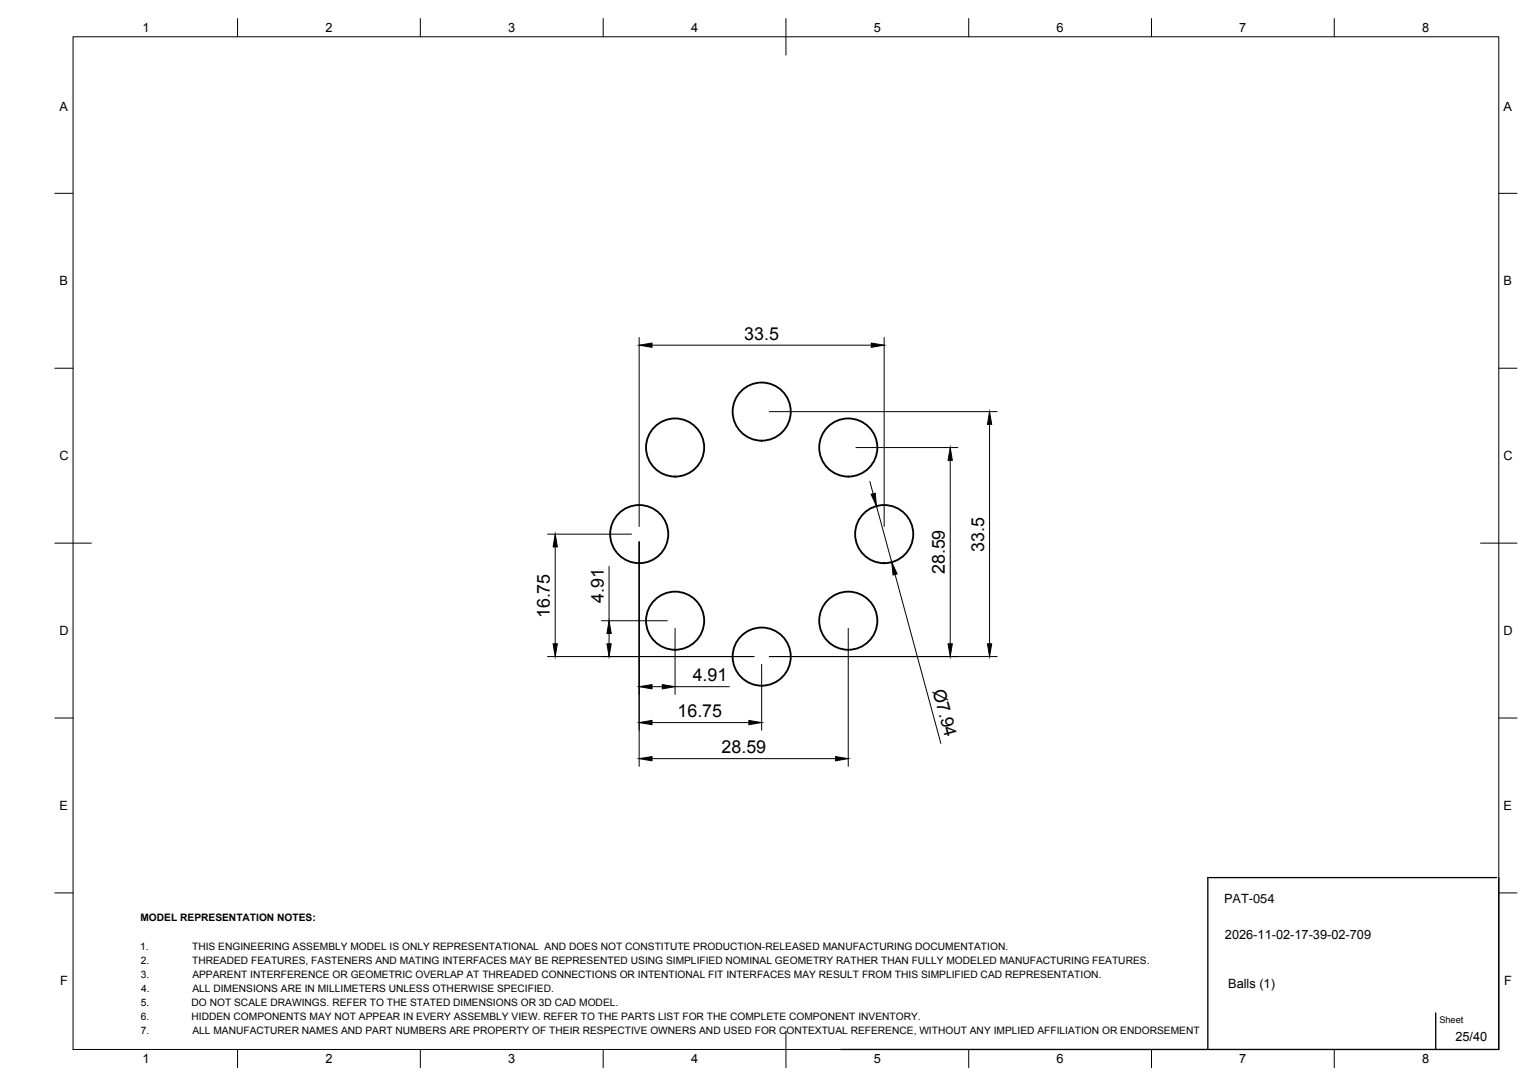
ISO-10303-21;
HEADER;
/* Generated by software containing ST-Developer
 * from STEP Tools, Inc. (www.steptools.com) 
 */

FILE_DESCRIPTION(
/* description */ ('PAT-054'),
/* implementation_level */ '2;1');

FILE_NAME(
/* name */ 'Balls (1).step',
/* time_stamp */ '2026-10-29T16:38:13-07:00',
/* author */ (''),
/* organization */ (''),
/* preprocessor_version */ 'ST-DEVELOPER v20.2',
/* originating_system */ 'Autodesk Translation Framework v15.17.0.0',
/* authorisation */ '');

FILE_SCHEMA (('AUTOMOTIVE_DESIGN { 1 0 10303 214 3 1 1 }'));
ENDSEC;

DATA;
#10=MECHANICAL_DESIGN_GEOMETRIC_PRESENTATION_REPRESENTATION('',(#922,#923,#924,#925,#926,#927,#928,#929),#33981);
#761=SPHERICAL_SURFACE('',#14041,0.3969);
#762=SPHERICAL_SURFACE('',#14043,0.3969);
#763=SPHERICAL_SURFACE('',#14045,0.3969);
#764=SPHERICAL_SURFACE('',#14047,0.3969);
#765=SPHERICAL_SURFACE('',#14049,0.3969);
#766=SPHERICAL_SURFACE('',#14051,0.3969);
#767=SPHERICAL_SURFACE('',#14053,0.3969);
#768=SPHERICAL_SURFACE('',#14055,0.3969);
#827=SHAPE_REPRESENTATION_RELATIONSHIP('SRR','None',#34202,#871);
#871=ADVANCED_BREP_SHAPE_REPRESENTATION('',(#981,#982,#983,#984,#985,#986,
#987,#988),#33950);
#922=STYLED_ITEM('',(#34517),#981);
#923=STYLED_ITEM('',(#34517),#982);
#924=STYLED_ITEM('',(#34517),#983);
#925=STYLED_ITEM('',(#34517),#984);
#926=STYLED_ITEM('',(#34517),#985);
#927=STYLED_ITEM('',(#34517),#986);
#928=STYLED_ITEM('',(#34517),#987);
#929=STYLED_ITEM('',(#34517),#988);
#981=MANIFOLD_SOLID_BREP('Body1',#13033);
#982=MANIFOLD_SOLID_BREP('Body2',#13034);
#983=MANIFOLD_SOLID_BREP('Body3',#13035);
#984=MANIFOLD_SOLID_BREP('Body4',#13036);
#985=MANIFOLD_SOLID_BREP('Body5',#13037);
#986=MANIFOLD_SOLID_BREP('Body6',#13038);
#987=MANIFOLD_SOLID_BREP('Body7',#13039);
#988=MANIFOLD_SOLID_BREP('Body8',#13040);
#1792=FACE_OUTER_BOUND('',#2644,.T.);
#1793=FACE_OUTER_BOUND('',#2645,.T.);
#1794=FACE_OUTER_BOUND('',#2646,.T.);
#1795=FACE_OUTER_BOUND('',#2647,.T.);
#1796=FACE_OUTER_BOUND('',#2648,.T.);
#1797=FACE_OUTER_BOUND('',#2649,.T.);
#1798=FACE_OUTER_BOUND('',#2650,.T.);
#1799=FACE_OUTER_BOUND('',#2651,.T.);
#2644=EDGE_LOOP('',(#9489,#9490));
#2645=EDGE_LOOP('',(#9491,#9492));
#2646=EDGE_LOOP('',(#9493,#9494));
#2647=EDGE_LOOP('',(#9495,#9496));
#2648=EDGE_LOOP('',(#9497,#9498));
#2649=EDGE_LOOP('',(#9499,#9500));
#2650=EDGE_LOOP('',(#9501,#9502));
#2651=EDGE_LOOP('',(#9503,#9504));
#5344=CIRCLE('',#14042,0.3969);
#5345=CIRCLE('',#14044,0.3969);
#5346=CIRCLE('',#14046,0.3969);
#5347=CIRCLE('',#14048,0.3969);
#5348=CIRCLE('',#14050,0.3969);
#5349=CIRCLE('',#14052,0.3969);
#5350=CIRCLE('',#14054,0.3969);
#5351=CIRCLE('',#14056,0.3969);
#5910=VERTEX_POINT('',#19864);
#5911=VERTEX_POINT('',#19865);
#5912=VERTEX_POINT('',#19868);
#5913=VERTEX_POINT('',#19869);
#5914=VERTEX_POINT('',#19872);
#5915=VERTEX_POINT('',#19873);
#5916=VERTEX_POINT('',#19876);
#5917=VERTEX_POINT('',#19877);
#5918=VERTEX_POINT('',#19880);
#5919=VERTEX_POINT('',#19881);
#5920=VERTEX_POINT('',#19884);
#5921=VERTEX_POINT('',#19885);
#5922=VERTEX_POINT('',#19888);
#5923=VERTEX_POINT('',#19889);
#5924=VERTEX_POINT('',#19892);
#5925=VERTEX_POINT('',#19893);
#7244=EDGE_CURVE('',#5910,#5911,#5344,.T.);
#7245=EDGE_CURVE('',#5912,#5913,#5345,.T.);
#7246=EDGE_CURVE('',#5914,#5915,#5346,.T.);
#7247=EDGE_CURVE('',#5916,#5917,#5347,.T.);
#7248=EDGE_CURVE('',#5918,#5919,#5348,.T.);
#7249=EDGE_CURVE('',#5920,#5921,#5349,.T.);
#7250=EDGE_CURVE('',#5922,#5923,#5350,.T.);
#7251=EDGE_CURVE('',#5924,#5925,#5351,.T.);
#9489=ORIENTED_EDGE('',*,*,#7244,.T.);
#9490=ORIENTED_EDGE('',*,*,#7244,.F.);
#9491=ORIENTED_EDGE('',*,*,#7245,.T.);
#9492=ORIENTED_EDGE('',*,*,#7245,.F.);
#9493=ORIENTED_EDGE('',*,*,#7246,.T.);
#9494=ORIENTED_EDGE('',*,*,#7246,.F.);
#9495=ORIENTED_EDGE('',*,*,#7247,.T.);
#9496=ORIENTED_EDGE('',*,*,#7247,.F.);
#9497=ORIENTED_EDGE('',*,*,#7248,.T.);
#9498=ORIENTED_EDGE('',*,*,#7248,.F.);
#9499=ORIENTED_EDGE('',*,*,#7249,.T.);
#9500=ORIENTED_EDGE('',*,*,#7249,.F.);
#9501=ORIENTED_EDGE('',*,*,#7250,.T.);
#9502=ORIENTED_EDGE('',*,*,#7250,.F.);
#9503=ORIENTED_EDGE('',*,*,#7251,.T.);
#9504=ORIENTED_EDGE('',*,*,#7251,.F.);
#12504=ADVANCED_FACE('',(#1792),#761,.T.);
#12505=ADVANCED_FACE('',(#1793),#762,.T.);
#12506=ADVANCED_FACE('',(#1794),#763,.T.);
#12507=ADVANCED_FACE('',(#1795),#764,.T.);
#12508=ADVANCED_FACE('',(#1796),#765,.T.);
#12509=ADVANCED_FACE('',(#1797),#766,.T.);
#12510=ADVANCED_FACE('',(#1798),#767,.T.);
#12511=ADVANCED_FACE('',(#1799),#768,.T.);
#13033=CLOSED_SHELL('',(#12504));
#13034=CLOSED_SHELL('',(#12505));
#13035=CLOSED_SHELL('',(#12506));
#13036=CLOSED_SHELL('',(#12507));
#13037=CLOSED_SHELL('',(#12508));
#13038=CLOSED_SHELL('',(#12509));
#13039=CLOSED_SHELL('',(#12510));
#13040=CLOSED_SHELL('',(#12511));
#14040=AXIS2_PLACEMENT_3D('',#19862,#16099,#16100);
#14041=AXIS2_PLACEMENT_3D('',#19863,#16101,#16102);
#14042=AXIS2_PLACEMENT_3D('',#19866,#16103,#16104);
#14043=AXIS2_PLACEMENT_3D('',#19867,#16105,#16106);
#14044=AXIS2_PLACEMENT_3D('',#19870,#16107,#16108);
#14045=AXIS2_PLACEMENT_3D('',#19871,#16109,#16110);
#14046=AXIS2_PLACEMENT_3D('',#19874,#16111,#16112);
#14047=AXIS2_PLACEMENT_3D('',#19875,#16113,#16114);
#14048=AXIS2_PLACEMENT_3D('',#19878,#16115,#16116);
#14049=AXIS2_PLACEMENT_3D('',#19879,#16117,#16118);
#14050=AXIS2_PLACEMENT_3D('',#19882,#16119,#16120);
#14051=AXIS2_PLACEMENT_3D('',#19883,#16121,#16122);
#14052=AXIS2_PLACEMENT_3D('',#19886,#16123,#16124);
#14053=AXIS2_PLACEMENT_3D('',#19887,#16125,#16126);
#14054=AXIS2_PLACEMENT_3D('',#19890,#16127,#16128);
#14055=AXIS2_PLACEMENT_3D('',#19891,#16129,#16130);
#14056=AXIS2_PLACEMENT_3D('',#19894,#16131,#16132);
#16099=DIRECTION('axis',(0.,0.,1.));
#16100=DIRECTION('refdir',(1.,0.,0.));
#16101=DIRECTION('center_axis',(0.,0.,1.));
#16102=DIRECTION('ref_axis',(1.,0.,0.));
#16103=DIRECTION('center_axis',(1.22464679914735E-16,-1.,0.));
#16104=DIRECTION('ref_axis',(-1.,-1.22464679914735E-16,0.));
#16105=DIRECTION('center_axis',(0.707106781186548,0.,0.707106781186548));
#16106=DIRECTION('ref_axis',(0.707106781186548,0.,-0.707106781186548));
#16107=DIRECTION('center_axis',(8.65956056235493E-17,-1.,-8.65956056235493E-17));
#16108=DIRECTION('ref_axis',(-0.707106781186548,-1.22464679914735E-16,0.707106781186548));
#16109=DIRECTION('center_axis',(1.,0.,0.));
#16110=DIRECTION('ref_axis',(6.12323399573677E-17,0.,-1.));
#16111=DIRECTION('center_axis',(7.49879891330929E-33,-1.,-1.22464679914735E-16));
#16112=DIRECTION('ref_axis',(-6.12323399573677E-17,-1.22464679914735E-16,
1.));
#16113=DIRECTION('center_axis',(0.707106781186548,0.,-0.707106781186548));
#16114=DIRECTION('ref_axis',(-0.707106781186548,0.,-0.707106781186548));
#16115=DIRECTION('center_axis',(-8.65956056235493E-17,-1.,-8.65956056235493E-17));
#16116=DIRECTION('ref_axis',(0.707106781186548,-1.22464679914735E-16,0.707106781186548));
#16117=DIRECTION('center_axis',(0.,0.,-1.));
#16118=DIRECTION('ref_axis',(-1.,0.,-1.22464679914735E-16));
#16119=DIRECTION('center_axis',(-1.22464679914735E-16,-1.,-1.49975978266186E-32));
#16120=DIRECTION('ref_axis',(1.,-1.22464679914735E-16,1.22464679914735E-16));
#16121=DIRECTION('center_axis',(-0.707106781186548,0.,-0.707106781186548));
#16122=DIRECTION('ref_axis',(-0.707106781186548,0.,0.707106781186548));
#16123=DIRECTION('center_axis',(-8.65956056235493E-17,-1.,8.65956056235493E-17));
#16124=DIRECTION('ref_axis',(0.707106781186548,-1.22464679914735E-16,-0.707106781186548));
#16125=DIRECTION('center_axis',(-1.,0.,0.));
#16126=DIRECTION('ref_axis',(-1.83697019872103E-16,0.,1.));
#16127=DIRECTION('center_axis',(-2.24963967399279E-32,-1.,1.22464679914735E-16));
#16128=DIRECTION('ref_axis',(1.83697019872103E-16,-1.22464679914735E-16,
-1.));
#16129=DIRECTION('center_axis',(-0.707106781186548,0.,0.707106781186548));
#16130=DIRECTION('ref_axis',(0.707106781186548,0.,0.707106781186548));
#16131=DIRECTION('center_axis',(8.65956056235493E-17,-1.,8.65956056235494E-17));
#16132=DIRECTION('ref_axis',(-0.707106781186548,-1.22464679914735E-16,-0.707106781186548));
#19862=CARTESIAN_POINT('',(0.,0.,0.));
#19863=CARTESIAN_POINT('Origin',(1.675,0.,0.));
#19864=CARTESIAN_POINT('',(1.675,-2.97627328869245E-33,0.3969));
#19865=CARTESIAN_POINT('',(1.675,-2.97627328869245E-33,-0.3969));
#19866=CARTESIAN_POINT('Origin',(1.675,0.,0.));
#19867=CARTESIAN_POINT('Origin',(1.18440385848747,0.,-1.18440385848747));
#19868=CARTESIAN_POINT('',(1.46505453994041,3.1867025333467E-33,-0.903753177034526));
#19869=CARTESIAN_POINT('',(0.903753177034527,-9.13924911073161E-33,-1.46505453994041));
#19870=CARTESIAN_POINT('Origin',(1.18440385848747,0.,-1.18440385848747));
#19871=CARTESIAN_POINT('Origin',(1.02564169428591E-16,0.,-1.675));
#19872=CARTESIAN_POINT('',(0.3969,-2.97627328869246E-33,-1.675));
#19873=CARTESIAN_POINT('',(-0.3969,-2.97627328869245E-33,-1.675));
#19874=CARTESIAN_POINT('Origin',(1.02564169428591E-16,0.,-1.675));
#19875=CARTESIAN_POINT('Origin',(-1.18440385848747,0.,-1.18440385848747));
#19876=CARTESIAN_POINT('',(-0.903753177034526,3.1867025333467E-33,-1.46505453994041));
#19877=CARTESIAN_POINT('',(-1.46505453994041,-9.13924911073161E-33,-0.903753177034527));
#19878=CARTESIAN_POINT('Origin',(-1.18440385848747,0.,-1.18440385848747));
#19879=CARTESIAN_POINT('Origin',(-1.675,0.,-2.05128338857182E-16));
#19880=CARTESIAN_POINT('',(-1.675,-2.97627328869246E-33,-0.3969));
#19881=CARTESIAN_POINT('',(-1.675,-2.97627328869245E-33,0.3969));
#19882=CARTESIAN_POINT('Origin',(-1.675,0.,-2.05128338857182E-16));
#19883=CARTESIAN_POINT('Origin',(-1.18440385848747,0.,1.18440385848747));
#19884=CARTESIAN_POINT('',(-1.46505453994041,6.26819044436628E-33,0.903753177034526));
#19885=CARTESIAN_POINT('',(-0.903753177034527,-1.22207370217512E-32,1.46505453994041));
#19886=CARTESIAN_POINT('Origin',(-1.18440385848747,0.,1.18440385848747));
#19887=CARTESIAN_POINT('Origin',(-3.07692508285772E-16,0.,1.675));
#19888=CARTESIAN_POINT('',(-0.3969,-2.97627328869246E-33,1.675));
#19889=CARTESIAN_POINT('',(0.396899999999999,-2.97627328869245E-33,1.675));
#19890=CARTESIAN_POINT('Origin',(-3.07692508285772E-16,0.,1.675));
#19891=CARTESIAN_POINT('Origin',(1.18440385848747,0.,1.18440385848747));
#19892=CARTESIAN_POINT('',(0.903753177034526,9.34967835538585E-33,1.46505453994041));
#19893=CARTESIAN_POINT('',(1.46505453994041,-1.53022249327708E-32,0.903753177034527));
#19894=CARTESIAN_POINT('Origin',(1.18440385848747,0.,1.18440385848747));
#33898=UNCERTAINTY_MEASURE_WITH_UNIT(LENGTH_MEASURE(0.001),#33982,
'DISTANCE_ACCURACY_VALUE',
'Maximum model space distance between geometric entities at asserted c
onnectivities');
#33929=UNCERTAINTY_MEASURE_WITH_UNIT(LENGTH_MEASURE(0.001),#33982,
'DISTANCE_ACCURACY_VALUE',
'Maximum model space distance between geometric entities at asserted c
onnectivities');
#33950=(
GEOMETRIC_REPRESENTATION_CONTEXT(3)
GLOBAL_UNCERTAINTY_ASSIGNED_CONTEXT((#33898))
GLOBAL_UNIT_ASSIGNED_CONTEXT((#33982,#33984,#33985))
REPRESENTATION_CONTEXT('','3D')
);
#33981=(
GEOMETRIC_REPRESENTATION_CONTEXT(3)
GLOBAL_UNCERTAINTY_ASSIGNED_CONTEXT((#33929))
GLOBAL_UNIT_ASSIGNED_CONTEXT((#33982,#33984,#33985))
REPRESENTATION_CONTEXT('','3D')
);
#33982=(
LENGTH_UNIT()
NAMED_UNIT(*)
SI_UNIT(.CENTI.,.METRE.)
);
#33984=(
NAMED_UNIT(*)
PLANE_ANGLE_UNIT()
SI_UNIT($,.RADIAN.)
);
#33985=(
NAMED_UNIT(*)
SI_UNIT($,.STERADIAN.)
SOLID_ANGLE_UNIT()
);
#34006=SHAPE_DEFINITION_REPRESENTATION(#34062,#34202);
#34062=PRODUCT_DEFINITION_SHAPE('',$,#34254);
#34202=SHAPE_REPRESENTATION('',(#14040),#33950);
#34233=PRODUCT_DEFINITION_CONTEXT('part definition',#34388,'design');
#34254=PRODUCT_DEFINITION('Balls (1)','Balls (1)',#34305,#34233);
#34305=PRODUCT_DEFINITION_FORMATION('',$,#34410);
#34388=APPLICATION_CONTEXT(
'Core Data for Automotive Mechanical Design Process');
#34389=PRODUCT_CONTEXT('part definition',#34388,'mechanical');
#34410=PRODUCT('Balls (1)','Balls (1)','Balls (1)',(#34389));
#34511=COLOUR_RGB('Grey',0.48,0.52,0.57);
#34512=FILL_AREA_STYLE_COLOUR('',#34511);
#34513=FILL_AREA_STYLE('',(#34512));
#34514=SURFACE_STYLE_FILL_AREA(#34513);
#34515=SURFACE_SIDE_STYLE('',(#34514));
#34516=SURFACE_STYLE_USAGE(.BOTH.,#34515);
#34517=PRESENTATION_STYLE_ASSIGNMENT((#34516));
ENDSEC;
END-ISO-10303-21;
